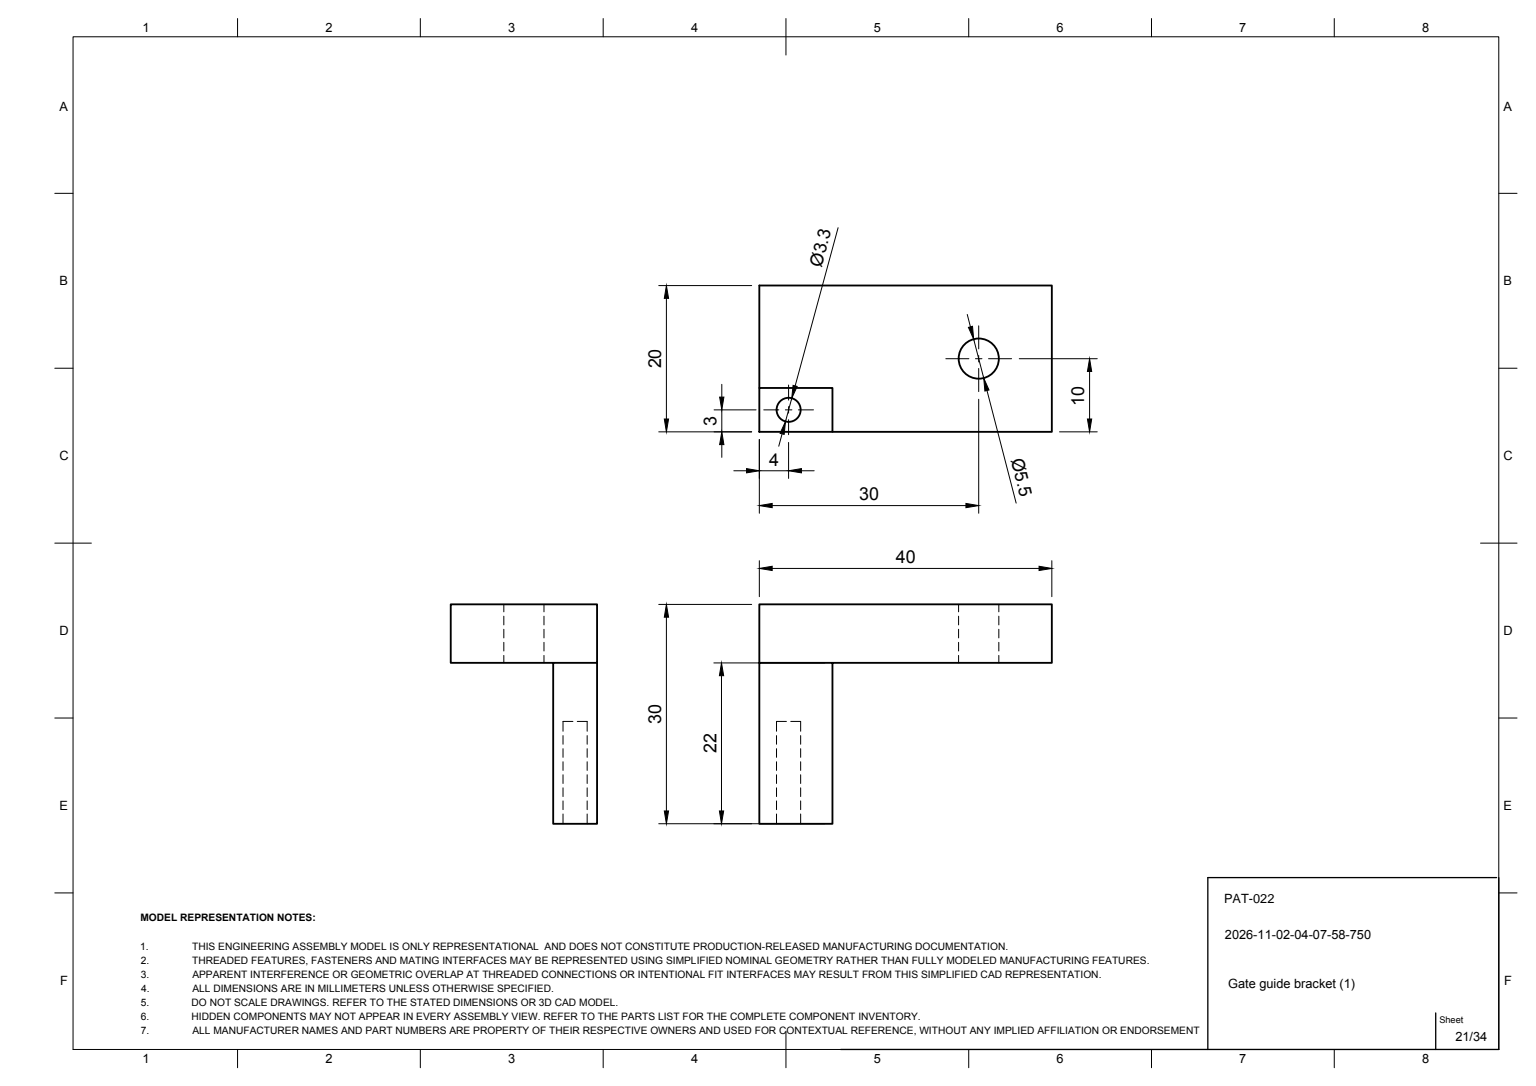
ISO-10303-21;
HEADER;
/* Generated by software containing ST-Developer
 * from STEP Tools, Inc. (www.steptools.com) 
 */

FILE_DESCRIPTION(
/* description */ ('Chute with adjustable gate'),
/* implementation_level */ '2;1');

FILE_NAME(
/* name */ 'Gate guide bracket (1).step',
/* time_stamp */ '2026-10-27T10:52:28-07:00',
/* author */ (''),
/* organization */ (''),
/* preprocessor_version */ 'ST-DEVELOPER v20.2',
/* originating_system */ 'Autodesk Translation Framework v15.17.0.0',
/* authorisation */ '');

FILE_SCHEMA (('AUTOMOTIVE_DESIGN { 1 0 10303 214 3 1 1 }'));
ENDSEC;

DATA;
#10=MECHANICAL_DESIGN_GEOMETRIC_PRESENTATION_REPRESENTATION('',(#430),#13094);
#366=SHAPE_REPRESENTATION_RELATIONSHIP('SRR','None',#13267,#398);
#398=ADVANCED_BREP_SHAPE_REPRESENTATION('',(#462),#13076);
#430=STYLED_ITEM('',(#13474),#462);
#462=MANIFOLD_SOLID_BREP('Body1',#7613);
#543=FACE_BOUND('',#1561,.T.);
#544=FACE_BOUND('',#1566,.T.);
#545=FACE_BOUND('',#1569,.T.);
#712=PLANE('',#8238);
#713=PLANE('',#8242);
#714=PLANE('',#8243);
#715=PLANE('',#8244);
#716=PLANE('',#8245);
#717=PLANE('',#8246);
#718=PLANE('',#8247);
#719=PLANE('',#8248);
#720=PLANE('',#8249);
#721=PLANE('',#8250);
#1072=FACE_OUTER_BOUND('',#1556,.T.);
#1073=FACE_OUTER_BOUND('',#1557,.T.);
#1074=FACE_OUTER_BOUND('',#1558,.T.);
#1075=FACE_OUTER_BOUND('',#1559,.T.);
#1076=FACE_OUTER_BOUND('',#1560,.T.);
#1077=FACE_OUTER_BOUND('',#1562,.T.);
#1078=FACE_OUTER_BOUND('',#1563,.T.);
#1079=FACE_OUTER_BOUND('',#1564,.T.);
#1080=FACE_OUTER_BOUND('',#1565,.T.);
#1081=FACE_OUTER_BOUND('',#1567,.T.);
#1082=FACE_OUTER_BOUND('',#1568,.T.);
#1083=FACE_OUTER_BOUND('',#1570,.T.);
#1556=EDGE_LOOP('',(#5888,#5889,#5890,#5891));
#1557=EDGE_LOOP('',(#5892));
#1558=EDGE_LOOP('',(#5893,#5894,#5895,#5896));
#1559=EDGE_LOOP('',(#5897,#5898,#5899,#5900));
#1560=EDGE_LOOP('',(#5901,#5902,#5903,#5904));
#1561=EDGE_LOOP('',(#5905));
#1562=EDGE_LOOP('',(#5906,#5907,#5908,#5909));
#1563=EDGE_LOOP('',(#5910,#5911,#5912,#5913,#5914,#5915));
#1564=EDGE_LOOP('',(#5916,#5917,#5918,#5919,#5920,#5921));
#1565=EDGE_LOOP('',(#5922,#5923,#5924,#5925));
#1566=EDGE_LOOP('',(#5926));
#1567=EDGE_LOOP('',(#5927,#5928,#5929,#5930));
#1568=EDGE_LOOP('',(#5931,#5932,#5933,#5934,#5935,#5936));
#1569=EDGE_LOOP('',(#5937));
#1570=EDGE_LOOP('',(#5938,#5939,#5940,#5941));
#2139=LINE('',#11665,#2916);
#2140=LINE('',#11672,#2917);
#2141=LINE('',#11677,#2918);
#2142=LINE('',#11679,#2919);
#2143=LINE('',#11681,#2920);
#2144=LINE('',#11682,#2921);
#2145=LINE('',#11685,#2922);
#2146=LINE('',#11687,#2923);
#2147=LINE('',#11688,#2924);
#2148=LINE('',#11691,#2925);
#2149=LINE('',#11692,#2926);
#2150=LINE('',#11695,#2927);
#2151=LINE('',#11697,#2928);
#2152=LINE('',#11699,#2929);
#2153=LINE('',#11700,#2930);
#2154=LINE('',#11703,#2931);
#2155=LINE('',#11705,#2932);
#2156=LINE('',#11706,#2933);
#2157=LINE('',#11709,#2934);
#2158=LINE('',#11710,#2935);
#2159=LINE('',#11713,#2936);
#2160=LINE('',#11714,#2937);
#2161=LINE('',#11716,#2938);
#2916=VECTOR('',#9479,0.164999999999999);
#2917=VECTOR('',#9488,0.274999999999999);
#2918=VECTOR('',#9493,1.);
#2919=VECTOR('',#9494,1.);
#2920=VECTOR('',#9495,1.);
#2921=VECTOR('',#9496,1.);
#2922=VECTOR('',#9499,1.);
#2923=VECTOR('',#9500,1.);
#2924=VECTOR('',#9501,1.);
#2925=VECTOR('',#9504,1.);
#2926=VECTOR('',#9505,1.);
#2927=VECTOR('',#9508,1.);
#2928=VECTOR('',#9509,1.);
#2929=VECTOR('',#9510,1.);
#2930=VECTOR('',#9511,1.);
#2931=VECTOR('',#9514,1.);
#2932=VECTOR('',#9515,1.);
#2933=VECTOR('',#9516,1.);
#2934=VECTOR('',#9519,1.);
#2935=VECTOR('',#9520,1.);
#2936=VECTOR('',#9523,1.);
#2937=VECTOR('',#9524,1.);
#2938=VECTOR('',#9527,1.);
#3486=CIRCLE('',#8236,0.164999999999999);
#3487=CIRCLE('',#8237,0.164999999999999);
#3488=CIRCLE('',#8240,0.274999999999999);
#3489=CIRCLE('',#8241,0.274999999999999);
#3827=VERTEX_POINT('',#11662);
#3828=VERTEX_POINT('',#11664);
#3829=VERTEX_POINT('',#11669);
#3830=VERTEX_POINT('',#11671);
#3831=VERTEX_POINT('',#11675);
#3832=VERTEX_POINT('',#11676);
#3833=VERTEX_POINT('',#11678);
#3834=VERTEX_POINT('',#11680);
#3835=VERTEX_POINT('',#11684);
#3836=VERTEX_POINT('',#11686);
#3837=VERTEX_POINT('',#11690);
#3838=VERTEX_POINT('',#11694);
#3839=VERTEX_POINT('',#11696);
#3840=VERTEX_POINT('',#11698);
#3841=VERTEX_POINT('',#11702);
#3842=VERTEX_POINT('',#11704);
#3843=VERTEX_POINT('',#11708);
#3844=VERTEX_POINT('',#11712);
#4577=EDGE_CURVE('',#3827,#3827,#3486,.T.);
#4578=EDGE_CURVE('',#3827,#3828,#2139,.T.);
#4579=EDGE_CURVE('',#3828,#3828,#3487,.T.);
#4580=EDGE_CURVE('',#3829,#3829,#3488,.T.);
#4581=EDGE_CURVE('',#3829,#3830,#2140,.T.);
#4582=EDGE_CURVE('',#3830,#3830,#3489,.T.);
#4583=EDGE_CURVE('',#3831,#3832,#2141,.T.);
#4584=EDGE_CURVE('',#3833,#3831,#2142,.T.);
#4585=EDGE_CURVE('',#3834,#3833,#2143,.T.);
#4586=EDGE_CURVE('',#3832,#3834,#2144,.T.);
#4587=EDGE_CURVE('',#3834,#3835,#2145,.T.);
#4588=EDGE_CURVE('',#3836,#3833,#2146,.T.);
#4589=EDGE_CURVE('',#3835,#3836,#2147,.T.);
#4590=EDGE_CURVE('',#3832,#3837,#2148,.T.);
#4591=EDGE_CURVE('',#3835,#3837,#2149,.T.);
#4592=EDGE_CURVE('',#3831,#3838,#2150,.T.);
#4593=EDGE_CURVE('',#3839,#3838,#2151,.T.);
#4594=EDGE_CURVE('',#3840,#3839,#2152,.T.);
#4595=EDGE_CURVE('',#3840,#3836,#2153,.T.);
#4596=EDGE_CURVE('',#3841,#3840,#2154,.T.);
#4597=EDGE_CURVE('',#3842,#3841,#2155,.T.);
#4598=EDGE_CURVE('',#3837,#3842,#2156,.T.);
#4599=EDGE_CURVE('',#3843,#3839,#2157,.T.);
#4600=EDGE_CURVE('',#3841,#3843,#2158,.T.);
#4601=EDGE_CURVE('',#3844,#3843,#2159,.T.);
#4602=EDGE_CURVE('',#3842,#3844,#2160,.T.);
#4603=EDGE_CURVE('',#3838,#3844,#2161,.T.);
#5888=ORIENTED_EDGE('',*,*,#4577,.F.);
#5889=ORIENTED_EDGE('',*,*,#4578,.T.);
#5890=ORIENTED_EDGE('',*,*,#4579,.T.);
#5891=ORIENTED_EDGE('',*,*,#4578,.F.);
#5892=ORIENTED_EDGE('',*,*,#4579,.F.);
#5893=ORIENTED_EDGE('',*,*,#4580,.F.);
#5894=ORIENTED_EDGE('',*,*,#4581,.T.);
#5895=ORIENTED_EDGE('',*,*,#4582,.F.);
#5896=ORIENTED_EDGE('',*,*,#4581,.F.);
#5897=ORIENTED_EDGE('',*,*,#4583,.F.);
#5898=ORIENTED_EDGE('',*,*,#4584,.F.);
#5899=ORIENTED_EDGE('',*,*,#4585,.F.);
#5900=ORIENTED_EDGE('',*,*,#4586,.F.);
#5901=ORIENTED_EDGE('',*,*,#4587,.F.);
#5902=ORIENTED_EDGE('',*,*,#4585,.T.);
#5903=ORIENTED_EDGE('',*,*,#4588,.F.);
#5904=ORIENTED_EDGE('',*,*,#4589,.F.);
#5905=ORIENTED_EDGE('',*,*,#4577,.T.);
#5906=ORIENTED_EDGE('',*,*,#4590,.F.);
#5907=ORIENTED_EDGE('',*,*,#4586,.T.);
#5908=ORIENTED_EDGE('',*,*,#4587,.T.);
#5909=ORIENTED_EDGE('',*,*,#4591,.T.);
#5910=ORIENTED_EDGE('',*,*,#4592,.T.);
#5911=ORIENTED_EDGE('',*,*,#4593,.F.);
#5912=ORIENTED_EDGE('',*,*,#4594,.F.);
#5913=ORIENTED_EDGE('',*,*,#4595,.T.);
#5914=ORIENTED_EDGE('',*,*,#4588,.T.);
#5915=ORIENTED_EDGE('',*,*,#4584,.T.);
#5916=ORIENTED_EDGE('',*,*,#4596,.F.);
#5917=ORIENTED_EDGE('',*,*,#4597,.F.);
#5918=ORIENTED_EDGE('',*,*,#4598,.F.);
#5919=ORIENTED_EDGE('',*,*,#4591,.F.);
#5920=ORIENTED_EDGE('',*,*,#4589,.T.);
#5921=ORIENTED_EDGE('',*,*,#4595,.F.);
#5922=ORIENTED_EDGE('',*,*,#4594,.T.);
#5923=ORIENTED_EDGE('',*,*,#4599,.F.);
#5924=ORIENTED_EDGE('',*,*,#4600,.F.);
#5925=ORIENTED_EDGE('',*,*,#4596,.T.);
#5926=ORIENTED_EDGE('',*,*,#4582,.T.);
#5927=ORIENTED_EDGE('',*,*,#4597,.T.);
#5928=ORIENTED_EDGE('',*,*,#4600,.T.);
#5929=ORIENTED_EDGE('',*,*,#4601,.F.);
#5930=ORIENTED_EDGE('',*,*,#4602,.F.);
#5931=ORIENTED_EDGE('',*,*,#4590,.T.);
#5932=ORIENTED_EDGE('',*,*,#4598,.T.);
#5933=ORIENTED_EDGE('',*,*,#4602,.T.);
#5934=ORIENTED_EDGE('',*,*,#4603,.F.);
#5935=ORIENTED_EDGE('',*,*,#4592,.F.);
#5936=ORIENTED_EDGE('',*,*,#4583,.T.);
#5937=ORIENTED_EDGE('',*,*,#4580,.T.);
#5938=ORIENTED_EDGE('',*,*,#4603,.T.);
#5939=ORIENTED_EDGE('',*,*,#4601,.T.);
#5940=ORIENTED_EDGE('',*,*,#4599,.T.);
#5941=ORIENTED_EDGE('',*,*,#4593,.T.);
#7142=CYLINDRICAL_SURFACE('',#8235,0.164999999999999);
#7143=CYLINDRICAL_SURFACE('',#8239,0.274999999999999);
#7340=ADVANCED_FACE('',(#1072),#7142,.F.);
#7341=ADVANCED_FACE('',(#1073),#712,.F.);
#7342=ADVANCED_FACE('',(#1074),#7143,.F.);
#7343=ADVANCED_FACE('',(#1075),#713,.T.);
#7344=ADVANCED_FACE('',(#1076,#543),#714,.T.);
#7345=ADVANCED_FACE('',(#1077),#715,.F.);
#7346=ADVANCED_FACE('',(#1078),#716,.T.);
#7347=ADVANCED_FACE('',(#1079),#717,.F.);
#7348=ADVANCED_FACE('',(#1080,#544),#718,.T.);
#7349=ADVANCED_FACE('',(#1081),#719,.T.);
#7350=ADVANCED_FACE('',(#1082,#545),#720,.T.);
#7351=ADVANCED_FACE('',(#1083),#721,.T.);
#7613=CLOSED_SHELL('',(#7340,#7341,#7342,#7343,#7344,#7345,#7346,#7347,
#7348,#7349,#7350,#7351));
#8234=AXIS2_PLACEMENT_3D('',#11660,#9473,#9474);
#8235=AXIS2_PLACEMENT_3D('',#11661,#9475,#9476);
#8236=AXIS2_PLACEMENT_3D('',#11663,#9477,#9478);
#8237=AXIS2_PLACEMENT_3D('',#11666,#9480,#9481);
#8238=AXIS2_PLACEMENT_3D('',#11667,#9482,#9483);
#8239=AXIS2_PLACEMENT_3D('',#11668,#9484,#9485);
#8240=AXIS2_PLACEMENT_3D('',#11670,#9486,#9487);
#8241=AXIS2_PLACEMENT_3D('',#11673,#9489,#9490);
#8242=AXIS2_PLACEMENT_3D('',#11674,#9491,#9492);
#8243=AXIS2_PLACEMENT_3D('',#11683,#9497,#9498);
#8244=AXIS2_PLACEMENT_3D('',#11689,#9502,#9503);
#8245=AXIS2_PLACEMENT_3D('',#11693,#9506,#9507);
#8246=AXIS2_PLACEMENT_3D('',#11701,#9512,#9513);
#8247=AXIS2_PLACEMENT_3D('',#11707,#9517,#9518);
#8248=AXIS2_PLACEMENT_3D('',#11711,#9521,#9522);
#8249=AXIS2_PLACEMENT_3D('',#11715,#9525,#9526);
#8250=AXIS2_PLACEMENT_3D('',#11717,#9528,#9529);
#9473=DIRECTION('axis',(0.,0.,1.));
#9474=DIRECTION('refdir',(1.,0.,0.));
#9475=DIRECTION('center_axis',(1.,0.,0.));
#9476=DIRECTION('ref_axis',(0.,0.,-1.));
#9477=DIRECTION('center_axis',(1.,0.,0.));
#9478=DIRECTION('ref_axis',(0.,0.,-1.));
#9479=DIRECTION('',(1.,0.,0.));
#9480=DIRECTION('center_axis',(1.,0.,0.));
#9481=DIRECTION('ref_axis',(0.,0.,-1.));
#9482=DIRECTION('center_axis',(1.,0.,0.));
#9483=DIRECTION('ref_axis',(0.,0.,-1.));
#9484=DIRECTION('center_axis',(1.,0.,0.));
#9485=DIRECTION('ref_axis',(0.,0.,-1.));
#9486=DIRECTION('center_axis',(1.,0.,0.));
#9487=DIRECTION('ref_axis',(0.,0.,-1.));
#9488=DIRECTION('',(1.,0.,0.));
#9489=DIRECTION('center_axis',(-1.,0.,0.));
#9490=DIRECTION('ref_axis',(0.,0.,-1.));
#9491=DIRECTION('center_axis',(0.,0.,1.));
#9492=DIRECTION('ref_axis',(1.,0.,0.));
#9493=DIRECTION('',(0.,-1.,0.));
#9494=DIRECTION('',(1.,0.,0.));
#9495=DIRECTION('',(0.,1.,0.));
#9496=DIRECTION('',(-1.,0.,0.));
#9497=DIRECTION('center_axis',(-1.,0.,0.));
#9498=DIRECTION('ref_axis',(0.,0.,1.));
#9499=DIRECTION('',(0.,0.,-1.));
#9500=DIRECTION('',(0.,0.,1.));
#9501=DIRECTION('',(0.,1.,0.));
#9502=DIRECTION('center_axis',(0.,1.,0.));
#9503=DIRECTION('ref_axis',(1.,0.,0.));
#9504=DIRECTION('',(0.,0.,-1.));
#9505=DIRECTION('',(1.,0.,0.));
#9506=DIRECTION('center_axis',(0.,1.,0.));
#9507=DIRECTION('ref_axis',(-1.,0.,0.));
#9508=DIRECTION('',(0.,0.,1.));
#9509=DIRECTION('',(-1.,0.,0.));
#9510=DIRECTION('',(0.,0.,1.));
#9511=DIRECTION('',(-1.,0.,0.));
#9512=DIRECTION('center_axis',(0.,0.,1.));
#9513=DIRECTION('ref_axis',(1.,0.,0.));
#9514=DIRECTION('',(0.,1.,0.));
#9515=DIRECTION('',(1.,0.,0.));
#9516=DIRECTION('',(0.,-1.,0.));
#9517=DIRECTION('center_axis',(1.,0.,0.));
#9518=DIRECTION('ref_axis',(0.,1.,0.));
#9519=DIRECTION('',(0.,1.,0.));
#9520=DIRECTION('',(0.,0.,1.));
#9521=DIRECTION('center_axis',(0.,-1.,0.));
#9522=DIRECTION('ref_axis',(1.,0.,0.));
#9523=DIRECTION('',(1.,0.,0.));
#9524=DIRECTION('',(0.,0.,1.));
#9525=DIRECTION('center_axis',(-1.,0.,0.));
#9526=DIRECTION('ref_axis',(0.,-1.,0.));
#9527=DIRECTION('',(0.,-1.,0.));
#9528=DIRECTION('center_axis',(0.,0.,1.));
#9529=DIRECTION('ref_axis',(1.,0.,0.));
#11660=CARTESIAN_POINT('',(0.,0.,0.));
#11661=CARTESIAN_POINT('Origin',(-1.1,-8.4,30.3));
#11662=CARTESIAN_POINT('',(-1.,-8.4,30.465));
#11663=CARTESIAN_POINT('Origin',(-1.,-8.4,30.3));
#11664=CARTESIAN_POINT('',(0.4,-8.4,30.465));
#11665=CARTESIAN_POINT('',(-1.1,-8.4,30.465));
#11666=CARTESIAN_POINT('Origin',(0.4,-8.4,30.3));
#11667=CARTESIAN_POINT('Origin',(0.4,-8.4,30.3));
#11668=CARTESIAN_POINT('Origin',(1.1,-11.,31.));
#11669=CARTESIAN_POINT('',(1.2,-11.,31.275));
#11670=CARTESIAN_POINT('Origin',(1.2,-11.,31.));
#11671=CARTESIAN_POINT('',(2.,-11.,31.275));
#11672=CARTESIAN_POINT('',(1.1,-11.,31.275));
#11673=CARTESIAN_POINT('Origin',(2.,-11.,31.));
#11674=CARTESIAN_POINT('Origin',(-1.,-9.,30.6));
#11675=CARTESIAN_POINT('',(1.2,-8.,30.6));
#11676=CARTESIAN_POINT('',(1.2,-9.,30.6));
#11677=CARTESIAN_POINT('',(1.2,-8.5,30.6));
#11678=CARTESIAN_POINT('',(-1.,-8.,30.6));
#11679=CARTESIAN_POINT('',(2.,-8.,30.6));
#11680=CARTESIAN_POINT('',(-1.,-9.,30.6));
#11681=CARTESIAN_POINT('',(-1.,-9.,30.6));
#11682=CARTESIAN_POINT('',(2.,-9.,30.6));
#11683=CARTESIAN_POINT('Origin',(-1.,-9.,30.));
#11684=CARTESIAN_POINT('',(-1.,-9.,30.));
#11685=CARTESIAN_POINT('',(-1.,-9.,30.6));
#11686=CARTESIAN_POINT('',(-1.,-8.,30.));
#11687=CARTESIAN_POINT('',(-1.,-8.,30.6));
#11688=CARTESIAN_POINT('',(-1.,-9.,30.));
#11689=CARTESIAN_POINT('Origin',(0.5,-9.,30.3));
#11690=CARTESIAN_POINT('',(1.2,-9.,30.));
#11691=CARTESIAN_POINT('',(1.2,-9.,30.15));
#11692=CARTESIAN_POINT('',(-1.,-9.,30.));
#11693=CARTESIAN_POINT('Origin',(2.,-8.,30.));
#11694=CARTESIAN_POINT('',(1.2,-8.,32.));
#11695=CARTESIAN_POINT('',(1.2,-8.,30.));
#11696=CARTESIAN_POINT('',(2.,-8.,32.));
#11697=CARTESIAN_POINT('',(2.,-8.,32.));
#11698=CARTESIAN_POINT('',(2.,-8.,30.));
#11699=CARTESIAN_POINT('',(2.,-8.,30.));
#11700=CARTESIAN_POINT('',(2.,-8.,30.));
#11701=CARTESIAN_POINT('Origin',(1.6,-10.,30.));
#11702=CARTESIAN_POINT('',(2.,-12.,30.));
#11703=CARTESIAN_POINT('',(2.,-12.,30.));
#11704=CARTESIAN_POINT('',(1.2,-12.,30.));
#11705=CARTESIAN_POINT('',(1.2,-12.,30.));
#11706=CARTESIAN_POINT('',(1.2,-8.,30.));
#11707=CARTESIAN_POINT('Origin',(2.,-12.,30.));
#11708=CARTESIAN_POINT('',(2.,-12.,32.));
#11709=CARTESIAN_POINT('',(2.,-12.,32.));
#11710=CARTESIAN_POINT('',(2.,-12.,30.));
#11711=CARTESIAN_POINT('Origin',(1.2,-12.,30.));
#11712=CARTESIAN_POINT('',(1.2,-12.,32.));
#11713=CARTESIAN_POINT('',(1.2,-12.,32.));
#11714=CARTESIAN_POINT('',(1.2,-12.,30.));
#11715=CARTESIAN_POINT('Origin',(1.2,-8.,30.));
#11716=CARTESIAN_POINT('',(1.2,-8.,32.));
#11717=CARTESIAN_POINT('Origin',(1.6,-10.,32.));
#13039=UNCERTAINTY_MEASURE_WITH_UNIT(LENGTH_MEASURE(0.001),#13095,
'DISTANCE_ACCURACY_VALUE',
'Maximum model space distance between geometric entities at asserted c
onnectivities');
#13057=UNCERTAINTY_MEASURE_WITH_UNIT(LENGTH_MEASURE(0.001),#13095,
'DISTANCE_ACCURACY_VALUE',
'Maximum model space distance between geometric entities at asserted c
onnectivities');
#13076=(
GEOMETRIC_REPRESENTATION_CONTEXT(3)
GLOBAL_UNCERTAINTY_ASSIGNED_CONTEXT((#13039))
GLOBAL_UNIT_ASSIGNED_CONTEXT((#13095,#13097,#13098))
REPRESENTATION_CONTEXT('','3D')
);
#13094=(
GEOMETRIC_REPRESENTATION_CONTEXT(3)
GLOBAL_UNCERTAINTY_ASSIGNED_CONTEXT((#13057))
GLOBAL_UNIT_ASSIGNED_CONTEXT((#13095,#13097,#13098))
REPRESENTATION_CONTEXT('','3D')
);
#13095=(
LENGTH_UNIT()
NAMED_UNIT(*)
SI_UNIT(.CENTI.,.METRE.)
);
#13097=(
NAMED_UNIT(*)
PLANE_ANGLE_UNIT()
SI_UNIT($,.RADIAN.)
);
#13098=(
NAMED_UNIT(*)
SI_UNIT($,.STERADIAN.)
SOLID_ANGLE_UNIT()
);
#13117=SHAPE_DEFINITION_REPRESENTATION(#13153,#13267);
#13153=PRODUCT_DEFINITION_SHAPE('',$,#13304);
#13267=SHAPE_REPRESENTATION('',(#8234),#13076);
#13285=PRODUCT_DEFINITION_CONTEXT('part definition',#13395,'design');
#13304=PRODUCT_DEFINITION('Gate guide bracket (1)',
'Gate guide bracket (1)',#13340,#13285);
#13340=PRODUCT_DEFINITION_FORMATION('',$,#13415);
#13395=APPLICATION_CONTEXT(
'Core Data for Automotive Mechanical Design Process');
#13396=PRODUCT_CONTEXT('part definition',#13395,'mechanical');
#13415=PRODUCT('Gate guide bracket (1)','Gate guide bracket (1)',
'Gate guide bracket (1)',(#13396));
#13468=COLOUR_RGB('Dark Blue',0.08,0.2,0.34);
#13469=FILL_AREA_STYLE_COLOUR('',#13468);
#13470=FILL_AREA_STYLE('',(#13469));
#13471=SURFACE_STYLE_FILL_AREA(#13470);
#13472=SURFACE_SIDE_STYLE('',(#13471));
#13473=SURFACE_STYLE_USAGE(.BOTH.,#13472);
#13474=PRESENTATION_STYLE_ASSIGNMENT((#13473));
ENDSEC;
END-ISO-10303-21;
